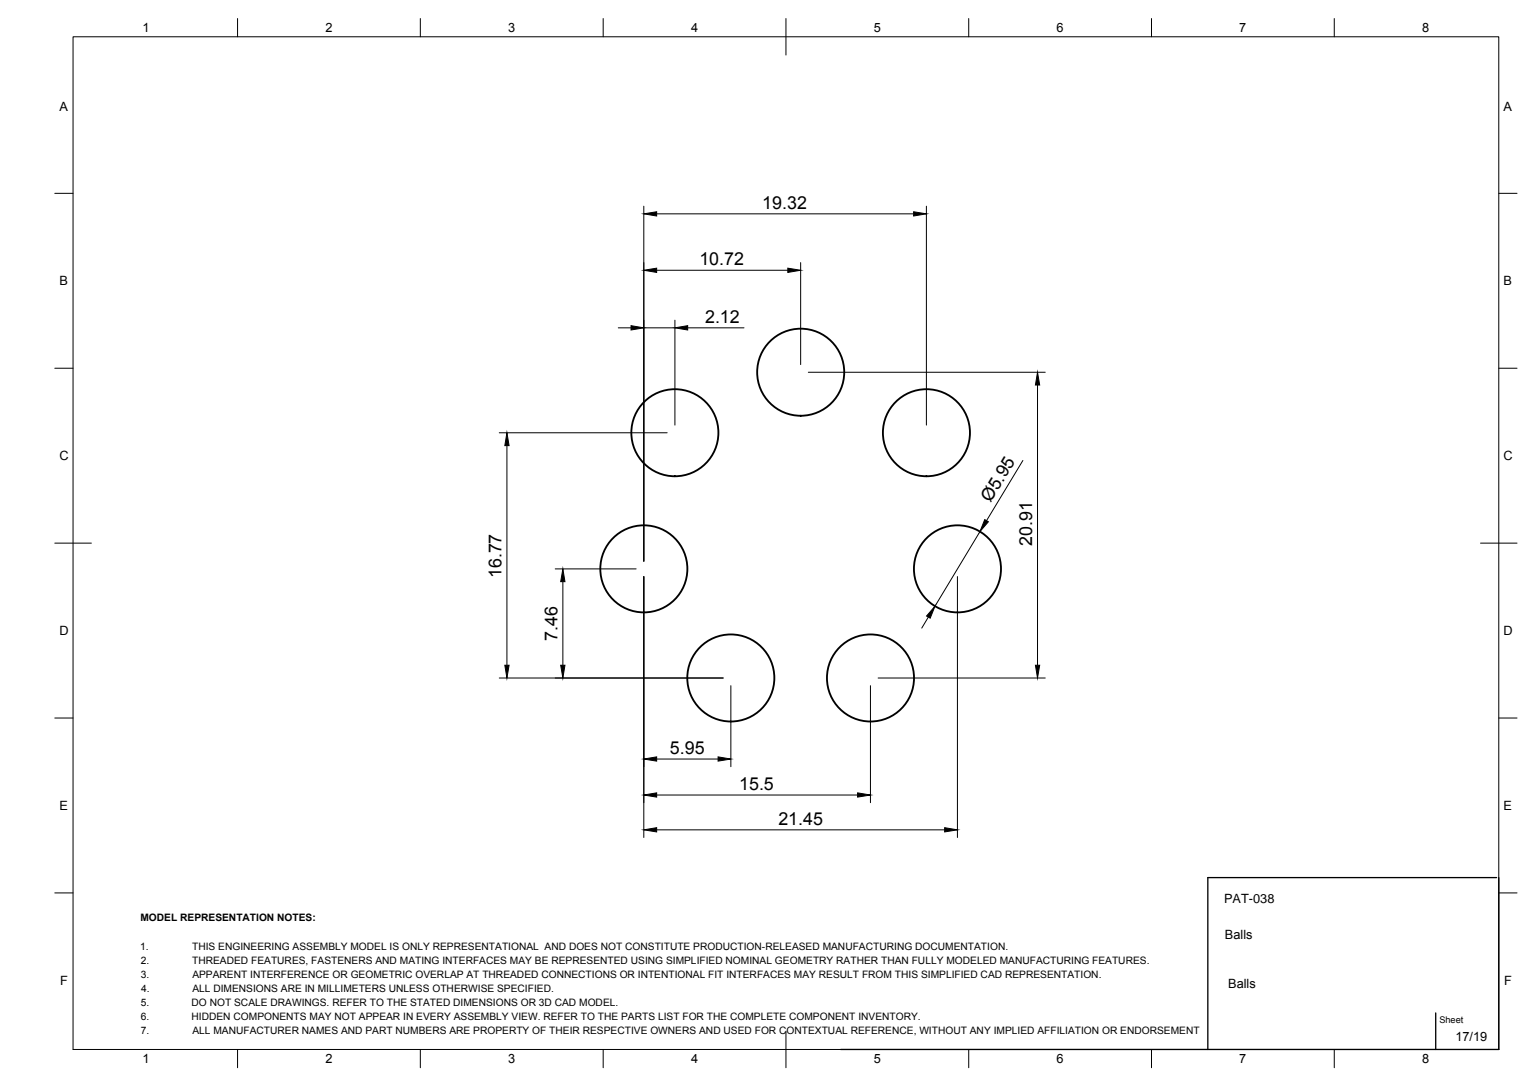
ISO-10303-21;
HEADER;
/* Generated by software containing ST-Developer
 * from STEP Tools, Inc. (www.steptools.com) 
 */

FILE_DESCRIPTION(
/* description */ ('Fork-mounted skate wheel'),
/* implementation_level */ '2;1');

FILE_NAME(
/* name */ 'Balls.step',
/* time_stamp */ '2026-10-29T16:11:26-07:00',
/* author */ (''),
/* organization */ (''),
/* preprocessor_version */ 'ST-DEVELOPER v20.2',
/* originating_system */ 'Autodesk Translation Framework v15.17.0.0',
/* authorisation */ '');

FILE_SCHEMA (('AUTOMOTIVE_DESIGN { 1 0 10303 214 3 1 1 }'));
ENDSEC;

DATA;
#10=MECHANICAL_DESIGN_GEOMETRIC_PRESENTATION_REPRESENTATION('',(#154,#155,#156,#157,#158,#159,#160),#3688);
#25=SPHERICAL_SURFACE('',#2119,0.29765);
#26=SPHERICAL_SURFACE('',#2121,0.29765);
#27=SPHERICAL_SURFACE('',#2123,0.29765);
#28=SPHERICAL_SURFACE('',#2125,0.29765);
#29=SPHERICAL_SURFACE('',#2127,0.29765);
#30=SPHERICAL_SURFACE('',#2129,0.29765);
#31=SPHERICAL_SURFACE('',#2131,0.29765);
#130=SHAPE_REPRESENTATION_RELATIONSHIP('SRR','None',#3755,#142);
#142=ADVANCED_BREP_SHAPE_REPRESENTATION('',(#172,#173,#174,#175,#176,#177,
#178),#3684);
#154=STYLED_ITEM('',(#3896),#172);
#155=STYLED_ITEM('',(#3896),#173);
#156=STYLED_ITEM('',(#3896),#174);
#157=STYLED_ITEM('',(#3896),#175);
#158=STYLED_ITEM('',(#3896),#176);
#159=STYLED_ITEM('',(#3896),#177);
#160=STYLED_ITEM('',(#3896),#178);
#172=MANIFOLD_SOLID_BREP('Body1',#1816);
#173=MANIFOLD_SOLID_BREP('Body2',#1817);
#174=MANIFOLD_SOLID_BREP('Body3',#1818);
#175=MANIFOLD_SOLID_BREP('Body4',#1819);
#176=MANIFOLD_SOLID_BREP('Body5',#1820);
#177=MANIFOLD_SOLID_BREP('Body6',#1821);
#178=MANIFOLD_SOLID_BREP('Body7',#1822);
#353=FACE_OUTER_BOUND('',#495,.T.);
#354=FACE_OUTER_BOUND('',#496,.T.);
#355=FACE_OUTER_BOUND('',#497,.T.);
#356=FACE_OUTER_BOUND('',#498,.T.);
#357=FACE_OUTER_BOUND('',#499,.T.);
#358=FACE_OUTER_BOUND('',#500,.T.);
#359=FACE_OUTER_BOUND('',#501,.T.);
#495=EDGE_LOOP('',(#1515,#1516));
#496=EDGE_LOOP('',(#1517,#1518));
#497=EDGE_LOOP('',(#1519,#1520));
#498=EDGE_LOOP('',(#1521,#1522));
#499=EDGE_LOOP('',(#1523,#1524));
#500=EDGE_LOOP('',(#1525,#1526));
#501=EDGE_LOOP('',(#1527,#1528));
#789=CIRCLE('',#2120,0.29765);
#790=CIRCLE('',#2122,0.29765);
#791=CIRCLE('',#2124,0.29765);
#792=CIRCLE('',#2126,0.29765);
#793=CIRCLE('',#2128,0.29765);
#794=CIRCLE('',#2130,0.29765);
#795=CIRCLE('',#2132,0.29765);
#937=VERTEX_POINT('',#3180);
#938=VERTEX_POINT('',#3181);
#939=VERTEX_POINT('',#3184);
#940=VERTEX_POINT('',#3185);
#941=VERTEX_POINT('',#3188);
#942=VERTEX_POINT('',#3189);
#943=VERTEX_POINT('',#3192);
#944=VERTEX_POINT('',#3193);
#945=VERTEX_POINT('',#3196);
#946=VERTEX_POINT('',#3197);
#947=VERTEX_POINT('',#3200);
#948=VERTEX_POINT('',#3201);
#949=VERTEX_POINT('',#3204);
#950=VERTEX_POINT('',#3205);
#1144=EDGE_CURVE('',#937,#938,#789,.T.);
#1145=EDGE_CURVE('',#939,#940,#790,.T.);
#1146=EDGE_CURVE('',#941,#942,#791,.T.);
#1147=EDGE_CURVE('',#943,#944,#792,.T.);
#1148=EDGE_CURVE('',#945,#946,#793,.T.);
#1149=EDGE_CURVE('',#947,#948,#794,.T.);
#1150=EDGE_CURVE('',#949,#950,#795,.T.);
#1515=ORIENTED_EDGE('',*,*,#1144,.T.);
#1516=ORIENTED_EDGE('',*,*,#1144,.F.);
#1517=ORIENTED_EDGE('',*,*,#1145,.T.);
#1518=ORIENTED_EDGE('',*,*,#1145,.F.);
#1519=ORIENTED_EDGE('',*,*,#1146,.T.);
#1520=ORIENTED_EDGE('',*,*,#1146,.F.);
#1521=ORIENTED_EDGE('',*,*,#1147,.T.);
#1522=ORIENTED_EDGE('',*,*,#1147,.F.);
#1523=ORIENTED_EDGE('',*,*,#1148,.T.);
#1524=ORIENTED_EDGE('',*,*,#1148,.F.);
#1525=ORIENTED_EDGE('',*,*,#1149,.T.);
#1526=ORIENTED_EDGE('',*,*,#1149,.F.);
#1527=ORIENTED_EDGE('',*,*,#1150,.T.);
#1528=ORIENTED_EDGE('',*,*,#1150,.F.);
#1771=ADVANCED_FACE('',(#353),#25,.T.);
#1772=ADVANCED_FACE('',(#354),#26,.T.);
#1773=ADVANCED_FACE('',(#355),#27,.T.);
#1774=ADVANCED_FACE('',(#356),#28,.T.);
#1775=ADVANCED_FACE('',(#357),#29,.T.);
#1776=ADVANCED_FACE('',(#358),#30,.T.);
#1777=ADVANCED_FACE('',(#359),#31,.T.);
#1816=CLOSED_SHELL('',(#1771));
#1817=CLOSED_SHELL('',(#1772));
#1818=CLOSED_SHELL('',(#1773));
#1819=CLOSED_SHELL('',(#1774));
#1820=CLOSED_SHELL('',(#1775));
#1821=CLOSED_SHELL('',(#1776));
#1822=CLOSED_SHELL('',(#1777));
#2118=AXIS2_PLACEMENT_3D('',#3178,#2623,#2624);
#2119=AXIS2_PLACEMENT_3D('',#3179,#2625,#2626);
#2120=AXIS2_PLACEMENT_3D('',#3182,#2627,#2628);
#2121=AXIS2_PLACEMENT_3D('',#3183,#2629,#2630);
#2122=AXIS2_PLACEMENT_3D('',#3186,#2631,#2632);
#2123=AXIS2_PLACEMENT_3D('',#3187,#2633,#2634);
#2124=AXIS2_PLACEMENT_3D('',#3190,#2635,#2636);
#2125=AXIS2_PLACEMENT_3D('',#3191,#2637,#2638);
#2126=AXIS2_PLACEMENT_3D('',#3194,#2639,#2640);
#2127=AXIS2_PLACEMENT_3D('',#3195,#2641,#2642);
#2128=AXIS2_PLACEMENT_3D('',#3198,#2643,#2644);
#2129=AXIS2_PLACEMENT_3D('',#3199,#2645,#2646);
#2130=AXIS2_PLACEMENT_3D('',#3202,#2647,#2648);
#2131=AXIS2_PLACEMENT_3D('',#3203,#2649,#2650);
#2132=AXIS2_PLACEMENT_3D('',#3206,#2651,#2652);
#2623=DIRECTION('axis',(0.,0.,1.));
#2624=DIRECTION('refdir',(1.,0.,0.));
#2625=DIRECTION('center_axis',(0.,0.,1.));
#2626=DIRECTION('ref_axis',(1.,0.,0.));
#2627=DIRECTION('center_axis',(1.22464679914735E-16,-1.,0.));
#2628=DIRECTION('ref_axis',(-1.,-1.22464679914735E-16,0.));
#2629=DIRECTION('center_axis',(0.78183148246803,0.,0.623489801858733));
#2630=DIRECTION('ref_axis',(0.623489801858734,0.,-0.78183148246803));
#2631=DIRECTION('center_axis',(7.63554790147315E-17,-1.,-9.57467422477103E-17));
#2632=DIRECTION('ref_axis',(-0.623489801858734,-1.22464679914735E-16,0.78183148246803));
#2633=DIRECTION('center_axis',(0.974927912181824,0.,-0.222520933956314));
#2634=DIRECTION('ref_axis',(-0.222520933956314,0.,-0.974927912181824));
#2635=DIRECTION('center_axis',(-2.7250954951288E-17,-1.,-1.19394234705288E-16));
#2636=DIRECTION('ref_axis',(0.222520933956314,-1.22464679914735E-16,0.974927912181824));
#2637=DIRECTION('center_axis',(0.433883739117558,0.,-0.900968867902419));
#2638=DIRECTION('ref_axis',(-0.900968867902419,0.,-0.433883739117558));
#2639=DIRECTION('center_axis',(-1.10336864020811E-16,-1.,-5.31354332312403E-17));
#2640=DIRECTION('ref_axis',(0.900968867902419,-1.22464679914735E-16,0.433883739117558));
#2641=DIRECTION('center_axis',(-0.433883739117558,0.,-0.900968867902419));
#2642=DIRECTION('ref_axis',(-0.900968867902419,0.,0.433883739117558));
#2643=DIRECTION('center_axis',(-1.10336864020811E-16,-1.,5.31354332312403E-17));
#2644=DIRECTION('ref_axis',(0.900968867902419,-1.22464679914735E-16,-0.433883739117558));
#2645=DIRECTION('center_axis',(-0.974927912181824,0.,-0.222520933956314));
#2646=DIRECTION('ref_axis',(-0.222520933956315,0.,0.974927912181824));
#2647=DIRECTION('center_axis',(-2.7250954951288E-17,-1.,1.19394234705288E-16));
#2648=DIRECTION('ref_axis',(0.222520933956315,-1.22464679914735E-16,-0.974927912181824));
#2649=DIRECTION('center_axis',(-0.78183148246803,0.,0.623489801858734));
#2650=DIRECTION('ref_axis',(0.623489801858733,0.,0.78183148246803));
#2651=DIRECTION('center_axis',(7.63554790147315E-17,-1.,9.57467422477103E-17));
#2652=DIRECTION('ref_axis',(-0.623489801858733,-1.22464679914735E-16,-0.78183148246803));
#3178=CARTESIAN_POINT('',(0.,0.,0.));
#3179=CARTESIAN_POINT('Origin',(1.1,0.,0.));
#3180=CARTESIAN_POINT('',(1.1,-2.23201749654651E-33,0.29765));
#3181=CARTESIAN_POINT('',(1.1,-2.23201749654651E-33,-0.29765));
#3182=CARTESIAN_POINT('Origin',(1.1,0.,0.));
#3183=CARTESIAN_POINT('Origin',(0.685838782044607,0.,-0.860014630714833));
#3184=CARTESIAN_POINT('',(0.918550922801216,-5.31350540756609E-33,-0.674432891191581));
#3185=CARTESIAN_POINT('',(0.453126641287998,8.49470414473068E-34,-1.04559637023808));
#3186=CARTESIAN_POINT('Origin',(0.685838782044607,0.,-0.860014630714833));
#3187=CARTESIAN_POINT('Origin',(-0.244773027351946,0.,-1.07242070340001));
#3188=CARTESIAN_POINT('',(0.0454142657089739,-2.23201749654651E-33,-1.1386540593921));
#3189=CARTESIAN_POINT('',(-0.534960320412865,-2.23201749654651E-33,-1.00618734740791));
#3190=CARTESIAN_POINT('Origin',(-0.244773027351946,0.,-1.07242070340001));
#3191=CARTESIAN_POINT('Origin',(-0.991065754692661,0.,-0.477272113029314));
#3192=CARTESIAN_POINT('',(-0.86192025974432,8.49470414473067E-34,-0.745445496560469));
#3193=CARTESIAN_POINT('',(-1.120211249641,-5.31350540756609E-33,-0.209098729498159));
#3194=CARTESIAN_POINT('Origin',(-0.991065754692661,0.,-0.477272113029314));
#3195=CARTESIAN_POINT('Origin',(-0.991065754692661,0.,0.477272113029314));
#3196=CARTESIAN_POINT('',(-1.120211249641,-2.23201749654651E-33,0.209098729498159));
#3197=CARTESIAN_POINT('',(-0.86192025974432,-2.23201749654651E-33,0.745445496560469));
#3198=CARTESIAN_POINT('Origin',(-0.991065754692661,0.,0.477272113029314));
#3199=CARTESIAN_POINT('Origin',(-0.244773027351946,0.,1.07242070340001));
#3200=CARTESIAN_POINT('',(-0.534960320412866,-2.23201749654651E-33,1.00618734740791));
#3201=CARTESIAN_POINT('',(0.0454142657089737,-2.23201749654651E-33,1.1386540593921));
#3202=CARTESIAN_POINT('Origin',(-0.244773027351946,0.,1.07242070340001));
#3203=CARTESIAN_POINT('Origin',(0.685838782044607,0.,0.860014630714833));
#3204=CARTESIAN_POINT('',(0.453126641287998,-2.23201749654651E-33,1.04559637023808));
#3205=CARTESIAN_POINT('',(0.918550922801216,-2.23201749654651E-33,0.674432891191581));
#3206=CARTESIAN_POINT('Origin',(0.685838782044607,0.,0.860014630714833));
#3667=UNCERTAINTY_MEASURE_WITH_UNIT(LENGTH_MEASURE(0.001),#3689,
'DISTANCE_ACCURACY_VALUE',
'Maximum model space distance between geometric entities at asserted c
onnectivities');
#3671=UNCERTAINTY_MEASURE_WITH_UNIT(LENGTH_MEASURE(0.001),#3689,
'DISTANCE_ACCURACY_VALUE',
'Maximum model space distance between geometric entities at asserted c
onnectivities');
#3684=(
GEOMETRIC_REPRESENTATION_CONTEXT(3)
GLOBAL_UNCERTAINTY_ASSIGNED_CONTEXT((#3667))
GLOBAL_UNIT_ASSIGNED_CONTEXT((#3689,#3691,#3692))
REPRESENTATION_CONTEXT('','3D')
);
#3688=(
GEOMETRIC_REPRESENTATION_CONTEXT(3)
GLOBAL_UNCERTAINTY_ASSIGNED_CONTEXT((#3671))
GLOBAL_UNIT_ASSIGNED_CONTEXT((#3689,#3691,#3692))
REPRESENTATION_CONTEXT('','3D')
);
#3689=(
LENGTH_UNIT()
NAMED_UNIT(*)
SI_UNIT(.CENTI.,.METRE.)
);
#3691=(
NAMED_UNIT(*)
PLANE_ANGLE_UNIT()
SI_UNIT($,.RADIAN.)
);
#3692=(
NAMED_UNIT(*)
SI_UNIT($,.STERADIAN.)
SOLID_ANGLE_UNIT()
);
#3705=SHAPE_DEFINITION_REPRESENTATION(#3727,#3755);
#3727=PRODUCT_DEFINITION_SHAPE('',$,#3772);
#3755=SHAPE_REPRESENTATION('',(#2118),#3684);
#3759=PRODUCT_DEFINITION_CONTEXT('part definition',#3809,'design');
#3772=PRODUCT_DEFINITION('Balls','Balls',#3788,#3759);
#3788=PRODUCT_DEFINITION_FORMATION('',$,#3823);
#3809=APPLICATION_CONTEXT(
'Core Data for Automotive Mechanical Design Process');
#3810=PRODUCT_CONTEXT('part definition',#3809,'mechanical');
#3823=PRODUCT('Balls','Balls','Balls',(#3810));
#3890=COLOUR_RGB('Grey',0.48,0.52,0.57);
#3891=FILL_AREA_STYLE_COLOUR('',#3890);
#3892=FILL_AREA_STYLE('',(#3891));
#3893=SURFACE_STYLE_FILL_AREA(#3892);
#3894=SURFACE_SIDE_STYLE('',(#3893));
#3895=SURFACE_STYLE_USAGE(.BOTH.,#3894);
#3896=PRESENTATION_STYLE_ASSIGNMENT((#3895));
ENDSEC;
END-ISO-10303-21;
